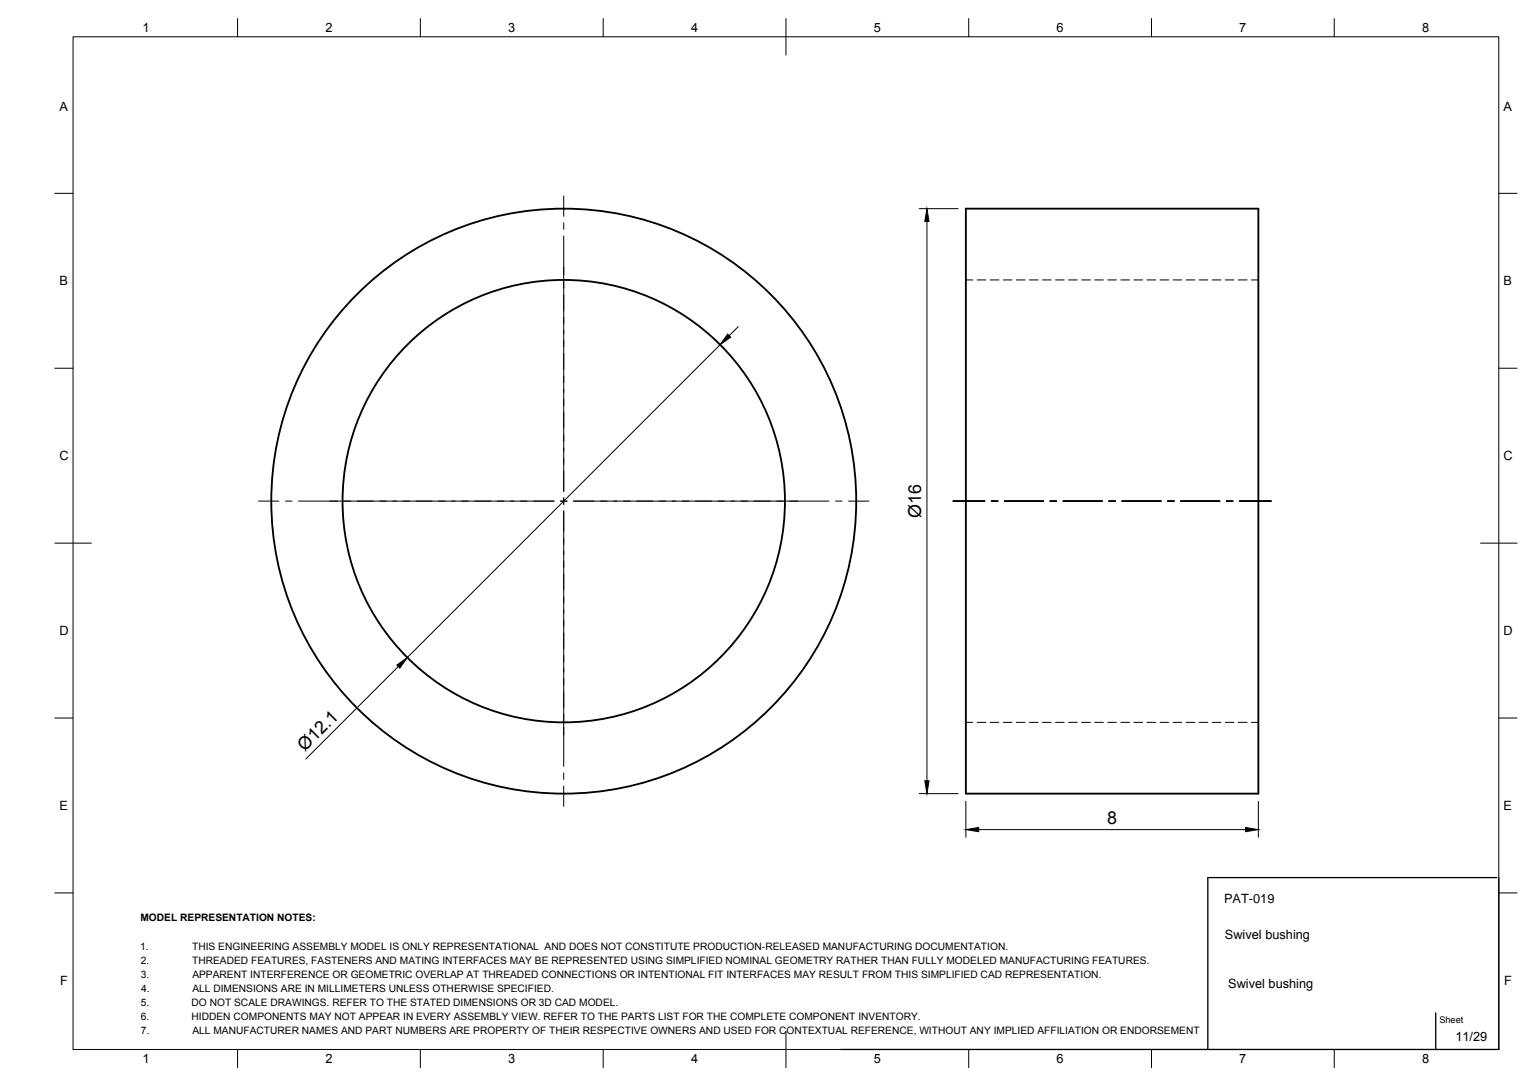
ISO-10303-21;
HEADER;
/* Generated by software containing ST-Developer
 * from STEP Tools, Inc. (www.steptools.com) 
 */

FILE_DESCRIPTION(
/* description */ ('Caster wheel assembly'),
/* implementation_level */ '2;1');

FILE_NAME(
/* name */ 'Swivel bushing.step',
/* time_stamp */ '2026-10-28T03:23:56-07:00',
/* author */ (''),
/* organization */ (''),
/* preprocessor_version */ 'ST-DEVELOPER v20.2',
/* originating_system */ 'Autodesk Translation Framework v15.17.0.0',
/* authorisation */ '');

FILE_SCHEMA (('AUTOMOTIVE_DESIGN { 1 0 10303 214 3 1 1 }'));
ENDSEC;

DATA;
#10=MECHANICAL_DESIGN_GEOMETRIC_PRESENTATION_REPRESENTATION('',(#228),#5385);
#184=SHAPE_REPRESENTATION_RELATIONSHIP('SRR','None',#5480,#206);
#206=ADVANCED_BREP_SHAPE_REPRESENTATION('',(#258),#5367);
#228=STYLED_ITEM('',(#5665),#258);
#258=MANIFOLD_SOLID_BREP('Body1',#2655);
#301=FACE_BOUND('',#666,.T.);
#302=FACE_BOUND('',#668,.T.);
#369=PLANE('',#3032);
#370=PLANE('',#3033);
#475=FACE_OUTER_BOUND('',#663,.T.);
#476=FACE_OUTER_BOUND('',#664,.T.);
#477=FACE_OUTER_BOUND('',#665,.T.);
#478=FACE_OUTER_BOUND('',#667,.T.);
#663=EDGE_LOOP('',(#2018,#2019,#2020,#2021));
#664=EDGE_LOOP('',(#2022,#2023,#2024,#2025));
#665=EDGE_LOOP('',(#2026));
#666=EDGE_LOOP('',(#2027));
#667=EDGE_LOOP('',(#2028));
#668=EDGE_LOOP('',(#2029));
#881=LINE('',#4493,#1015);
#882=LINE('',#4499,#1016);
#1015=VECTOR('',#3586,0.605);
#1016=VECTOR('',#3593,0.8);
#1111=CIRCLE('',#3027,0.605);
#1112=CIRCLE('',#3028,0.605);
#1113=CIRCLE('',#3030,0.8);
#1114=CIRCLE('',#3031,0.8);
#1314=VERTEX_POINT('',#4490);
#1315=VERTEX_POINT('',#4492);
#1316=VERTEX_POINT('',#4496);
#1317=VERTEX_POINT('',#4498);
#1577=EDGE_CURVE('',#1314,#1314,#1111,.T.);
#1578=EDGE_CURVE('',#1314,#1315,#881,.T.);
#1579=EDGE_CURVE('',#1315,#1315,#1112,.T.);
#1580=EDGE_CURVE('',#1316,#1316,#1113,.T.);
#1581=EDGE_CURVE('',#1316,#1317,#882,.T.);
#1582=EDGE_CURVE('',#1317,#1317,#1114,.T.);
#2018=ORIENTED_EDGE('',*,*,#1577,.F.);
#2019=ORIENTED_EDGE('',*,*,#1578,.T.);
#2020=ORIENTED_EDGE('',*,*,#1579,.T.);
#2021=ORIENTED_EDGE('',*,*,#1578,.F.);
#2022=ORIENTED_EDGE('',*,*,#1580,.F.);
#2023=ORIENTED_EDGE('',*,*,#1581,.T.);
#2024=ORIENTED_EDGE('',*,*,#1582,.T.);
#2025=ORIENTED_EDGE('',*,*,#1581,.F.);
#2026=ORIENTED_EDGE('',*,*,#1580,.T.);
#2027=ORIENTED_EDGE('',*,*,#1577,.T.);
#2028=ORIENTED_EDGE('',*,*,#1582,.F.);
#2029=ORIENTED_EDGE('',*,*,#1579,.F.);
#2444=CYLINDRICAL_SURFACE('',#3026,0.605);
#2445=CYLINDRICAL_SURFACE('',#3029,0.8);
#2535=ADVANCED_FACE('',(#475),#2444,.F.);
#2536=ADVANCED_FACE('',(#476),#2445,.T.);
#2537=ADVANCED_FACE('',(#477,#301),#369,.T.);
#2538=ADVANCED_FACE('',(#478,#302),#370,.F.);
#2655=CLOSED_SHELL('',(#2535,#2536,#2537,#2538));
#3025=AXIS2_PLACEMENT_3D('',#4488,#3580,#3581);
#3026=AXIS2_PLACEMENT_3D('',#4489,#3582,#3583);
#3027=AXIS2_PLACEMENT_3D('',#4491,#3584,#3585);
#3028=AXIS2_PLACEMENT_3D('',#4494,#3587,#3588);
#3029=AXIS2_PLACEMENT_3D('',#4495,#3589,#3590);
#3030=AXIS2_PLACEMENT_3D('',#4497,#3591,#3592);
#3031=AXIS2_PLACEMENT_3D('',#4500,#3594,#3595);
#3032=AXIS2_PLACEMENT_3D('',#4501,#3596,#3597);
#3033=AXIS2_PLACEMENT_3D('',#4502,#3598,#3599);
#3580=DIRECTION('axis',(0.,0.,1.));
#3581=DIRECTION('refdir',(1.,0.,0.));
#3582=DIRECTION('center_axis',(0.,0.,1.));
#3583=DIRECTION('ref_axis',(1.,0.,0.));
#3584=DIRECTION('center_axis',(0.,0.,-1.));
#3585=DIRECTION('ref_axis',(1.,0.,0.));
#3586=DIRECTION('',(0.,0.,-1.));
#3587=DIRECTION('center_axis',(0.,0.,-1.));
#3588=DIRECTION('ref_axis',(1.,0.,0.));
#3589=DIRECTION('center_axis',(0.,0.,1.));
#3590=DIRECTION('ref_axis',(1.,0.,0.));
#3591=DIRECTION('center_axis',(0.,0.,1.));
#3592=DIRECTION('ref_axis',(1.,0.,0.));
#3593=DIRECTION('',(0.,0.,-1.));
#3594=DIRECTION('center_axis',(0.,0.,1.));
#3595=DIRECTION('ref_axis',(1.,0.,0.));
#3596=DIRECTION('center_axis',(0.,0.,1.));
#3597=DIRECTION('ref_axis',(1.,0.,0.));
#3598=DIRECTION('center_axis',(0.,0.,1.));
#3599=DIRECTION('ref_axis',(1.,0.,0.));
#4488=CARTESIAN_POINT('',(0.,0.,0.));
#4489=CARTESIAN_POINT('Origin',(-2.,0.,8.5));
#4490=CARTESIAN_POINT('',(-2.605,-7.40911313484149E-17,9.3));
#4491=CARTESIAN_POINT('Origin',(-2.,0.,9.3));
#4492=CARTESIAN_POINT('',(-2.605,-7.40911313484149E-17,8.5));
#4493=CARTESIAN_POINT('',(-2.605,-7.40911313484149E-17,8.5));
#4494=CARTESIAN_POINT('Origin',(-2.,0.,8.5));
#4495=CARTESIAN_POINT('Origin',(-2.,0.,8.5));
#4496=CARTESIAN_POINT('',(-2.8,-9.79717439317883E-17,9.3));
#4497=CARTESIAN_POINT('Origin',(-2.,0.,9.3));
#4498=CARTESIAN_POINT('',(-2.8,-9.79717439317883E-17,8.5));
#4499=CARTESIAN_POINT('',(-2.8,-9.79717439317883E-17,8.5));
#4500=CARTESIAN_POINT('Origin',(-2.,0.,8.5));
#4501=CARTESIAN_POINT('Origin',(-2.,0.,9.3));
#4502=CARTESIAN_POINT('Origin',(-2.,0.,8.5));
#5339=UNCERTAINTY_MEASURE_WITH_UNIT(LENGTH_MEASURE(0.001),#5386,
'DISTANCE_ACCURACY_VALUE',
'Maximum model space distance between geometric entities at asserted c
onnectivities');
#5357=UNCERTAINTY_MEASURE_WITH_UNIT(LENGTH_MEASURE(0.001),#5386,
'DISTANCE_ACCURACY_VALUE',
'Maximum model space distance between geometric entities at asserted c
onnectivities');
#5367=(
GEOMETRIC_REPRESENTATION_CONTEXT(3)
GLOBAL_UNCERTAINTY_ASSIGNED_CONTEXT((#5339))
GLOBAL_UNIT_ASSIGNED_CONTEXT((#5386,#5388,#5389))
REPRESENTATION_CONTEXT('','3D')
);
#5385=(
GEOMETRIC_REPRESENTATION_CONTEXT(3)
GLOBAL_UNCERTAINTY_ASSIGNED_CONTEXT((#5357))
GLOBAL_UNIT_ASSIGNED_CONTEXT((#5386,#5388,#5389))
REPRESENTATION_CONTEXT('','3D')
);
#5386=(
LENGTH_UNIT()
NAMED_UNIT(*)
SI_UNIT(.CENTI.,.METRE.)
);
#5388=(
NAMED_UNIT(*)
PLANE_ANGLE_UNIT()
SI_UNIT($,.RADIAN.)
);
#5389=(
NAMED_UNIT(*)
SI_UNIT($,.STERADIAN.)
SOLID_ANGLE_UNIT()
);
#5399=SHAPE_DEFINITION_REPRESENTATION(#5431,#5480);
#5431=PRODUCT_DEFINITION_SHAPE('',$,#5508);
#5480=SHAPE_REPRESENTATION('',(#3025),#5367);
#5498=PRODUCT_DEFINITION_CONTEXT('part definition',#5581,'design');
#5508=PRODUCT_DEFINITION('Swivel bushing','Swivel bushing',#5535,#5498);
#5535=PRODUCT_DEFINITION_FORMATION('',$,#5592);
#5581=APPLICATION_CONTEXT(
'Core Data for Automotive Mechanical Design Process');
#5582=PRODUCT_CONTEXT('part definition',#5581,'mechanical');
#5592=PRODUCT('Swivel bushing','Swivel bushing','Swivel bushing',(#5582));
#5659=COLOUR_RGB('Sky Blue',0.24,0.69,0.87);
#5660=FILL_AREA_STYLE_COLOUR('',#5659);
#5661=FILL_AREA_STYLE('',(#5660));
#5662=SURFACE_STYLE_FILL_AREA(#5661);
#5663=SURFACE_SIDE_STYLE('',(#5662));
#5664=SURFACE_STYLE_USAGE(.BOTH.,#5663);
#5665=PRESENTATION_STYLE_ASSIGNMENT((#5664));
ENDSEC;
END-ISO-10303-21;
